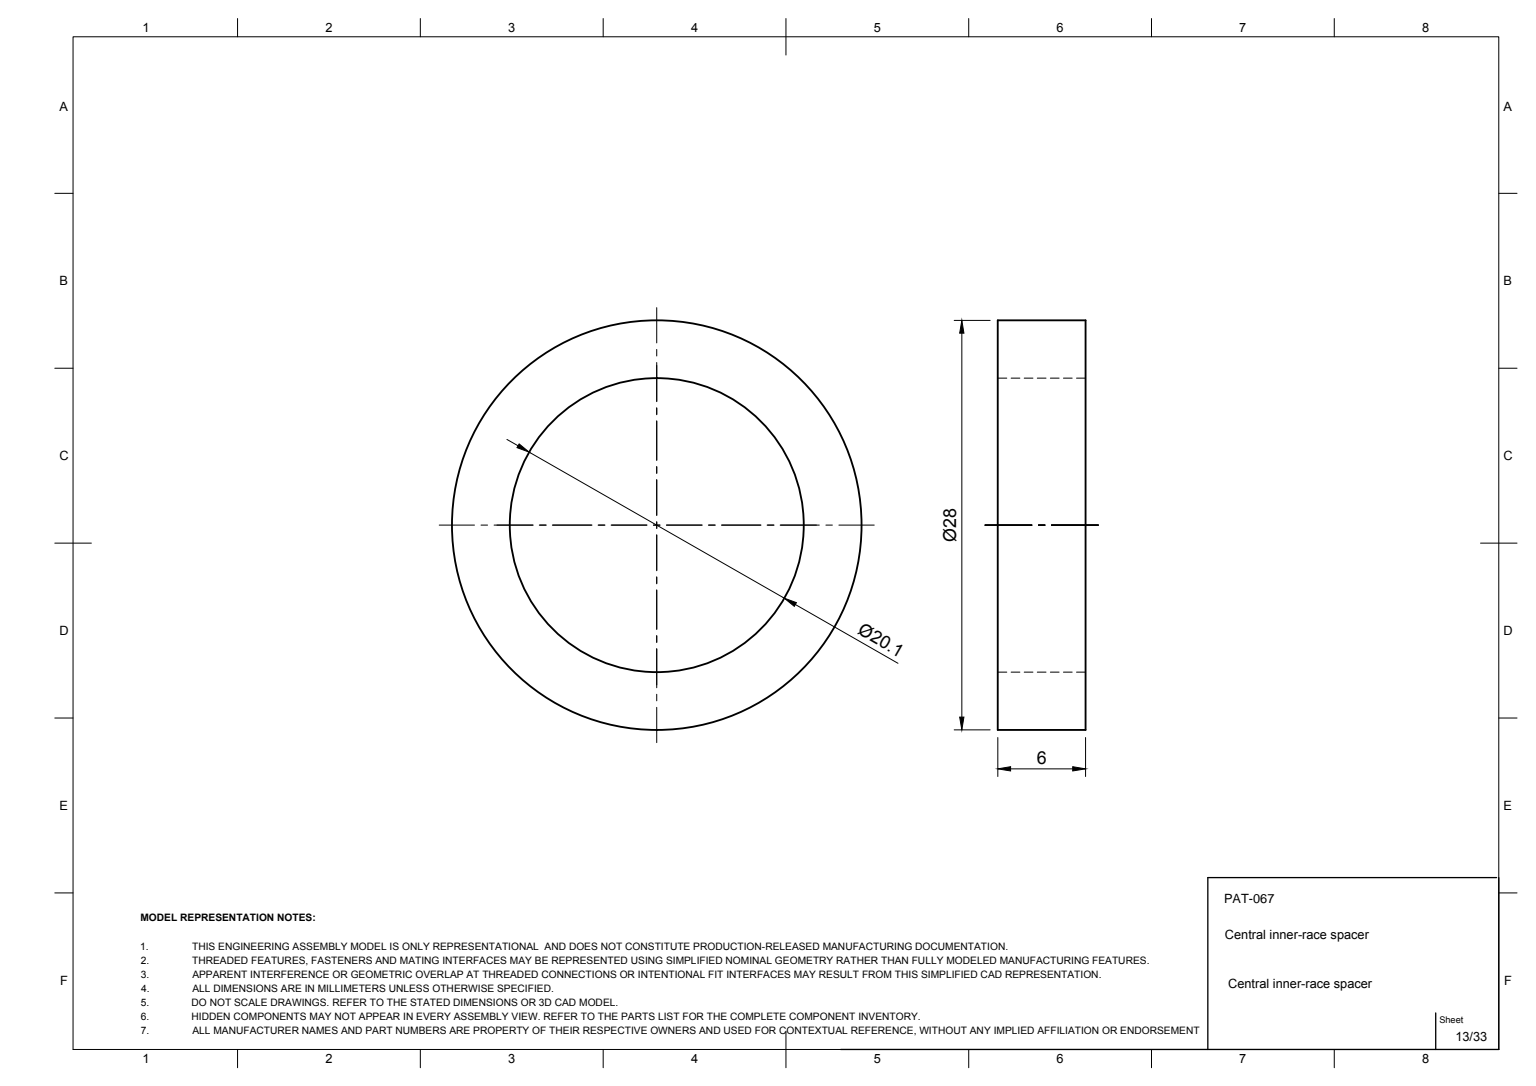
ISO-10303-21;
HEADER;
/* Generated by software containing ST-Developer
 * from STEP Tools, Inc. (www.steptools.com) 
 */

FILE_DESCRIPTION(
/* description */ ('Lifting hook block with sheave'),
/* implementation_level */ '2;1');

FILE_NAME(
/* name */ 'Central inner-race spacer.step',
/* time_stamp */ '2026-10-28T03:23:54-07:00',
/* author */ (''),
/* organization */ (''),
/* preprocessor_version */ 'ST-DEVELOPER v20.2',
/* originating_system */ 'Autodesk Translation Framework v15.17.0.0',
/* authorisation */ '');

FILE_SCHEMA (('AUTOMOTIVE_DESIGN { 1 0 10303 214 3 1 1 }'));
ENDSEC;

DATA;
#10=MECHANICAL_DESIGN_GEOMETRIC_PRESENTATION_REPRESENTATION('',(#359),#9391);
#299=SHAPE_REPRESENTATION_RELATIONSHIP('SRR','None',#9530,#329);
#329=ADVANCED_BREP_SHAPE_REPRESENTATION('',(#397),#9365);
#359=STYLED_ITEM('',(#9745),#397);
#397=MANIFOLD_SOLID_BREP('Body1',#4895);
#532=LINE('',#7994,#820);
#533=LINE('',#8000,#821);
#820=VECTOR('',#6419,1.005);
#821=VECTOR('',#6426,1.4);
#1040=CYLINDRICAL_SURFACE('',#5448,1.005);
#1041=CYLINDRICAL_SURFACE('',#5451,1.4);
#1151=FACE_BOUND('',#1640,.T.);
#1152=FACE_BOUND('',#1642,.T.);
#1304=FACE_OUTER_BOUND('',#1637,.T.);
#1305=FACE_OUTER_BOUND('',#1638,.T.);
#1306=FACE_OUTER_BOUND('',#1639,.T.);
#1307=FACE_OUTER_BOUND('',#1641,.T.);
#1637=EDGE_LOOP('',(#3638,#3639,#3640,#3641));
#1638=EDGE_LOOP('',(#3642,#3643,#3644,#3645));
#1639=EDGE_LOOP('',(#3646));
#1640=EDGE_LOOP('',(#3647));
#1641=EDGE_LOOP('',(#3648));
#1642=EDGE_LOOP('',(#3649));
#2011=CIRCLE('',#5449,1.005);
#2012=CIRCLE('',#5450,1.005);
#2013=CIRCLE('',#5452,1.4);
#2014=CIRCLE('',#5453,1.4);
#2344=VERTEX_POINT('',#7991);
#2345=VERTEX_POINT('',#7993);
#2346=VERTEX_POINT('',#7997);
#2347=VERTEX_POINT('',#7999);
#2823=EDGE_CURVE('',#2344,#2344,#2011,.T.);
#2824=EDGE_CURVE('',#2344,#2345,#532,.T.);
#2825=EDGE_CURVE('',#2345,#2345,#2012,.T.);
#2826=EDGE_CURVE('',#2346,#2346,#2013,.T.);
#2827=EDGE_CURVE('',#2346,#2347,#533,.T.);
#2828=EDGE_CURVE('',#2347,#2347,#2014,.T.);
#3638=ORIENTED_EDGE('',*,*,#2823,.F.);
#3639=ORIENTED_EDGE('',*,*,#2824,.T.);
#3640=ORIENTED_EDGE('',*,*,#2825,.T.);
#3641=ORIENTED_EDGE('',*,*,#2824,.F.);
#3642=ORIENTED_EDGE('',*,*,#2826,.F.);
#3643=ORIENTED_EDGE('',*,*,#2827,.T.);
#3644=ORIENTED_EDGE('',*,*,#2828,.T.);
#3645=ORIENTED_EDGE('',*,*,#2827,.F.);
#3646=ORIENTED_EDGE('',*,*,#2826,.T.);
#3647=ORIENTED_EDGE('',*,*,#2823,.T.);
#3648=ORIENTED_EDGE('',*,*,#2828,.F.);
#3649=ORIENTED_EDGE('',*,*,#2825,.F.);
#4494=PLANE('',#5454);
#4495=PLANE('',#5455);
#4680=ADVANCED_FACE('',(#1304),#1040,.F.);
#4681=ADVANCED_FACE('',(#1305),#1041,.T.);
#4682=ADVANCED_FACE('',(#1306,#1151),#4494,.T.);
#4683=ADVANCED_FACE('',(#1307,#1152),#4495,.F.);
#4895=CLOSED_SHELL('',(#4680,#4681,#4682,#4683));
#5447=AXIS2_PLACEMENT_3D('',#7989,#6413,#6414);
#5448=AXIS2_PLACEMENT_3D('',#7990,#6415,#6416);
#5449=AXIS2_PLACEMENT_3D('',#7992,#6417,#6418);
#5450=AXIS2_PLACEMENT_3D('',#7995,#6420,#6421);
#5451=AXIS2_PLACEMENT_3D('',#7996,#6422,#6423);
#5452=AXIS2_PLACEMENT_3D('',#7998,#6424,#6425);
#5453=AXIS2_PLACEMENT_3D('',#8001,#6427,#6428);
#5454=AXIS2_PLACEMENT_3D('',#8002,#6429,#6430);
#5455=AXIS2_PLACEMENT_3D('',#8003,#6431,#6432);
#6413=DIRECTION('axis',(0.,0.,1.));
#6414=DIRECTION('refdir',(1.,0.,0.));
#6415=DIRECTION('center_axis',(0.,1.,0.));
#6416=DIRECTION('ref_axis',(1.,0.,0.));
#6417=DIRECTION('center_axis',(0.,-1.,0.));
#6418=DIRECTION('ref_axis',(1.,0.,0.));
#6419=DIRECTION('',(0.,-1.,0.));
#6420=DIRECTION('center_axis',(0.,-1.,0.));
#6421=DIRECTION('ref_axis',(1.,0.,0.));
#6422=DIRECTION('center_axis',(0.,1.,0.));
#6423=DIRECTION('ref_axis',(1.,0.,0.));
#6424=DIRECTION('center_axis',(0.,1.,0.));
#6425=DIRECTION('ref_axis',(1.,0.,0.));
#6426=DIRECTION('',(0.,-1.,0.));
#6427=DIRECTION('center_axis',(0.,1.,0.));
#6428=DIRECTION('ref_axis',(1.,0.,0.));
#6429=DIRECTION('center_axis',(0.,1.,0.));
#6430=DIRECTION('ref_axis',(1.,0.,0.));
#6431=DIRECTION('center_axis',(0.,1.,0.));
#6432=DIRECTION('ref_axis',(1.,0.,0.));
#7989=CARTESIAN_POINT('',(0.,0.,0.));
#7990=CARTESIAN_POINT('Origin',(0.,-0.3,12.));
#7991=CARTESIAN_POINT('',(-1.005,0.3,12.));
#7992=CARTESIAN_POINT('Origin',(0.,0.3,12.));
#7993=CARTESIAN_POINT('',(-1.005,-0.3,12.));
#7994=CARTESIAN_POINT('',(-1.005,-0.3,12.));
#7995=CARTESIAN_POINT('Origin',(0.,-0.3,12.));
#7996=CARTESIAN_POINT('Origin',(0.,-0.3,12.));
#7997=CARTESIAN_POINT('',(-1.4,0.3,12.));
#7998=CARTESIAN_POINT('Origin',(0.,0.3,12.));
#7999=CARTESIAN_POINT('',(-1.4,-0.3,12.));
#8000=CARTESIAN_POINT('',(-1.4,-0.3,12.));
#8001=CARTESIAN_POINT('Origin',(0.,-0.3,12.));
#8002=CARTESIAN_POINT('Origin',(0.,0.3,12.));
#8003=CARTESIAN_POINT('Origin',(0.,-0.3,12.));
#9328=UNCERTAINTY_MEASURE_WITH_UNIT(LENGTH_MEASURE(0.001),#9392,
'DISTANCE_ACCURACY_VALUE',
'Maximum model space distance between geometric entities at asserted c
onnectivities');
#9354=UNCERTAINTY_MEASURE_WITH_UNIT(LENGTH_MEASURE(0.001),#9392,
'DISTANCE_ACCURACY_VALUE',
'Maximum model space distance between geometric entities at asserted c
onnectivities');
#9365=(
GEOMETRIC_REPRESENTATION_CONTEXT(3)
GLOBAL_UNCERTAINTY_ASSIGNED_CONTEXT((#9328))
GLOBAL_UNIT_ASSIGNED_CONTEXT((#9392,#9394,#9395))
REPRESENTATION_CONTEXT('','3D')
);
#9391=(
GEOMETRIC_REPRESENTATION_CONTEXT(3)
GLOBAL_UNCERTAINTY_ASSIGNED_CONTEXT((#9354))
GLOBAL_UNIT_ASSIGNED_CONTEXT((#9392,#9394,#9395))
REPRESENTATION_CONTEXT('','3D')
);
#9392=(
LENGTH_UNIT()
NAMED_UNIT(*)
SI_UNIT(.CENTI.,.METRE.)
);
#9394=(
NAMED_UNIT(*)
PLANE_ANGLE_UNIT()
SI_UNIT($,.RADIAN.)
);
#9395=(
NAMED_UNIT(*)
SI_UNIT($,.STERADIAN.)
SOLID_ANGLE_UNIT()
);
#9406=SHAPE_DEFINITION_REPRESENTATION(#9442,#9530);
#9442=PRODUCT_DEFINITION_SHAPE('',$,#9567);
#9530=SHAPE_REPRESENTATION('',(#5447),#9365);
#9556=PRODUCT_DEFINITION_CONTEXT('part definition',#9666,'design');
#9567=PRODUCT_DEFINITION('Central inner-race spacer',
'Central inner-race spacer',#9603,#9556);
#9603=PRODUCT_DEFINITION_FORMATION('',$,#9678);
#9666=APPLICATION_CONTEXT(
'Core Data for Automotive Mechanical Design Process');
#9667=PRODUCT_CONTEXT('part definition',#9666,'mechanical');
#9678=PRODUCT('Central inner-race spacer','Central inner-race spacer',
'Central inner-race spacer',(#9667));
#9739=COLOUR_RGB('Light Blue',0.38,0.62,0.78);
#9740=FILL_AREA_STYLE_COLOUR('',#9739);
#9741=FILL_AREA_STYLE('',(#9740));
#9742=SURFACE_STYLE_FILL_AREA(#9741);
#9743=SURFACE_SIDE_STYLE('',(#9742));
#9744=SURFACE_STYLE_USAGE(.BOTH.,#9743);
#9745=PRESENTATION_STYLE_ASSIGNMENT((#9744));
ENDSEC;
END-ISO-10303-21;
